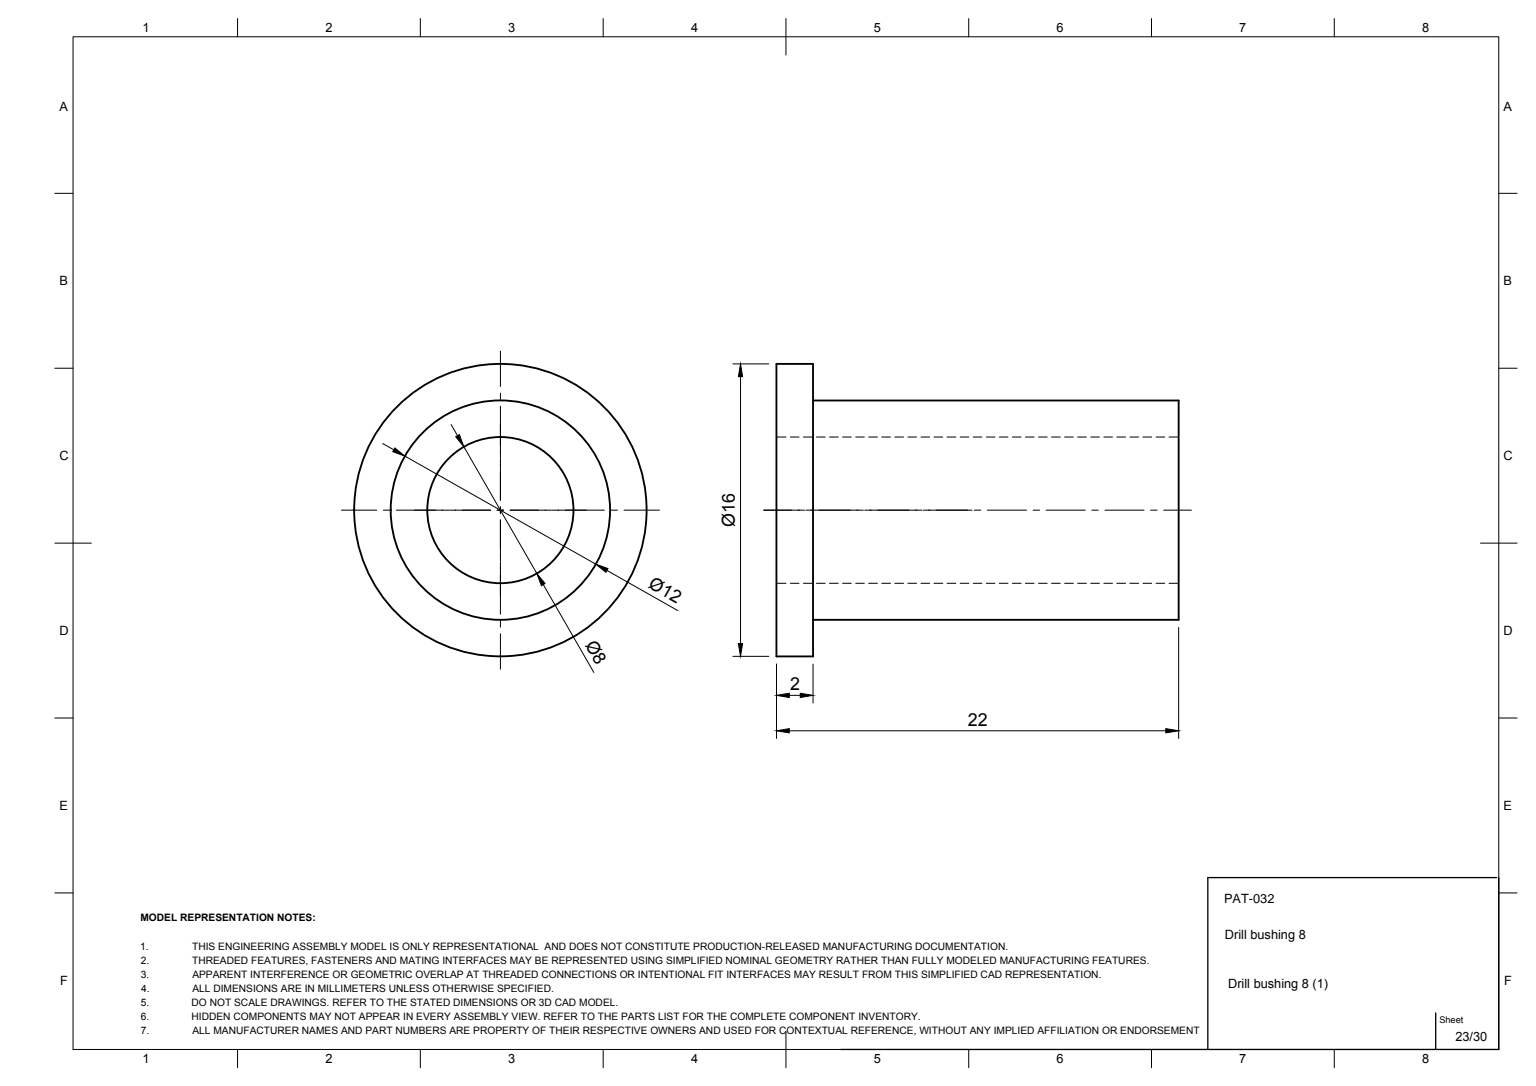
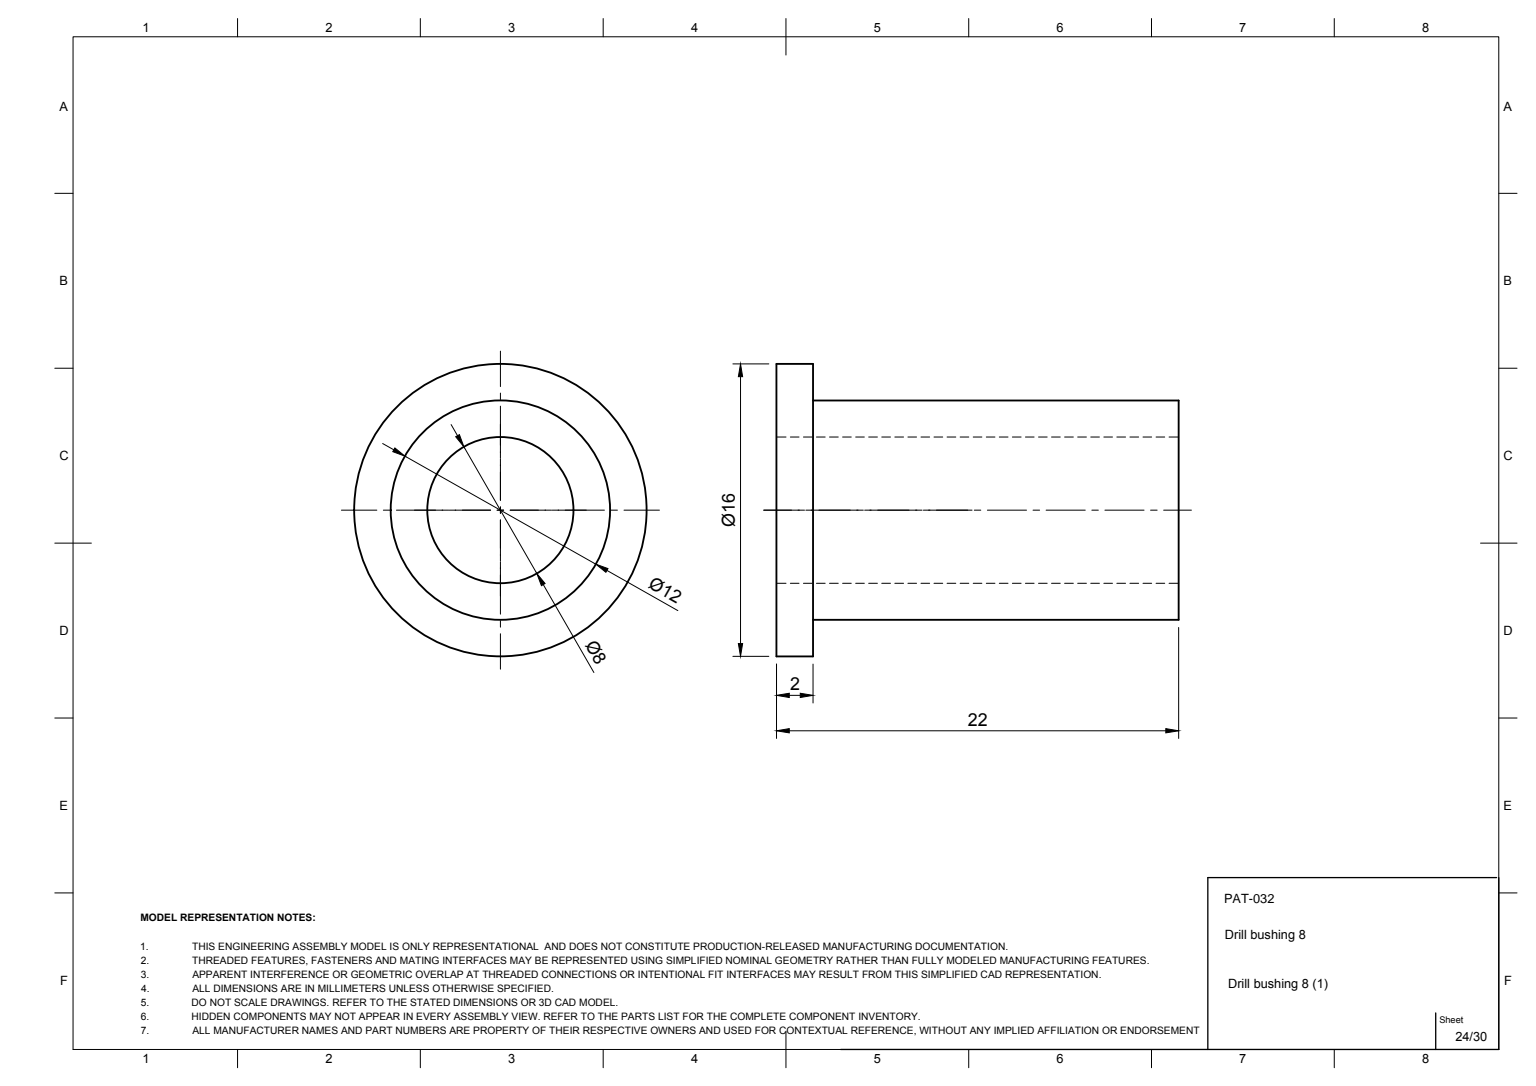
ISO-10303-21;
HEADER;
/* Generated by software containing ST-Developer
 * from STEP Tools, Inc. (www.steptools.com) 
 */

FILE_DESCRIPTION(
/* description */ ('Drill jig with bushing plate'),
/* implementation_level */ '2;1');

FILE_NAME(
/* name */ 'Drill bushing 8.step',
/* time_stamp */ '2026-10-27T10:51:08-07:00',
/* author */ (''),
/* organization */ (''),
/* preprocessor_version */ 'ST-DEVELOPER v20.2',
/* originating_system */ 'Autodesk Translation Framework v15.17.0.0',
/* authorisation */ '');

FILE_SCHEMA (('AUTOMOTIVE_DESIGN { 1 0 10303 214 3 1 1 }'));
ENDSEC;

DATA;
#10=MECHANICAL_DESIGN_GEOMETRIC_PRESENTATION_REPRESENTATION('',(#241),#6638);
#193=SHAPE_REPRESENTATION_RELATIONSHIP('SRR','None',#6758,#217);
#217=ADVANCED_BREP_SHAPE_REPRESENTATION('',(#263),#6631);
#241=STYLED_ITEM('',(#6957),#263);
#263=MANIFOLD_SOLID_BREP('Body1',#3610);
#355=FACE_BOUND('',#980,.T.);
#356=FACE_BOUND('',#983,.T.);
#357=FACE_BOUND('',#987,.T.);
#481=PLANE('',#4245);
#482=PLANE('',#4250);
#483=PLANE('',#4256);
#679=FACE_OUTER_BOUND('',#979,.T.);
#680=FACE_OUTER_BOUND('',#981,.T.);
#681=FACE_OUTER_BOUND('',#982,.T.);
#682=FACE_OUTER_BOUND('',#984,.T.);
#683=FACE_OUTER_BOUND('',#985,.T.);
#684=FACE_OUTER_BOUND('',#986,.T.);
#979=EDGE_LOOP('',(#3185));
#980=EDGE_LOOP('',(#3186));
#981=EDGE_LOOP('',(#3187,#3188,#3189,#3190));
#982=EDGE_LOOP('',(#3191));
#983=EDGE_LOOP('',(#3192));
#984=EDGE_LOOP('',(#3193,#3194,#3195,#3196));
#985=EDGE_LOOP('',(#3197,#3198,#3199,#3200));
#986=EDGE_LOOP('',(#3201));
#987=EDGE_LOOP('',(#3202));
#1266=LINE('',#6442,#1527);
#1267=LINE('',#6448,#1528);
#1268=LINE('',#6452,#1529);
#1527=VECTOR('',#5303,0.8);
#1528=VECTOR('',#5310,0.4);
#1529=VECTOR('',#5315,0.6);
#1688=CIRCLE('',#4246,0.8);
#1689=CIRCLE('',#4247,0.6);
#1690=CIRCLE('',#4249,0.8);
#1691=CIRCLE('',#4251,0.4);
#1692=CIRCLE('',#4253,0.4);
#1693=CIRCLE('',#4255,0.6);
#1968=VERTEX_POINT('',#6435);
#1969=VERTEX_POINT('',#6437);
#1970=VERTEX_POINT('',#6440);
#1971=VERTEX_POINT('',#6444);
#1972=VERTEX_POINT('',#6447);
#1973=VERTEX_POINT('',#6451);
#2380=EDGE_CURVE('',#1968,#1968,#1688,.T.);
#2381=EDGE_CURVE('',#1969,#1969,#1689,.T.);
#2382=EDGE_CURVE('',#1970,#1970,#1690,.T.);
#2383=EDGE_CURVE('',#1970,#1968,#1266,.T.);
#2384=EDGE_CURVE('',#1971,#1971,#1691,.T.);
#2385=EDGE_CURVE('',#1971,#1972,#1267,.T.);
#2386=EDGE_CURVE('',#1972,#1972,#1692,.T.);
#2387=EDGE_CURVE('',#1969,#1973,#1268,.T.);
#2388=EDGE_CURVE('',#1973,#1973,#1693,.T.);
#3185=ORIENTED_EDGE('',*,*,#2380,.F.);
#3186=ORIENTED_EDGE('',*,*,#2381,.T.);
#3187=ORIENTED_EDGE('',*,*,#2382,.F.);
#3188=ORIENTED_EDGE('',*,*,#2383,.T.);
#3189=ORIENTED_EDGE('',*,*,#2380,.T.);
#3190=ORIENTED_EDGE('',*,*,#2383,.F.);
#3191=ORIENTED_EDGE('',*,*,#2382,.T.);
#3192=ORIENTED_EDGE('',*,*,#2384,.T.);
#3193=ORIENTED_EDGE('',*,*,#2384,.F.);
#3194=ORIENTED_EDGE('',*,*,#2385,.T.);
#3195=ORIENTED_EDGE('',*,*,#2386,.T.);
#3196=ORIENTED_EDGE('',*,*,#2385,.F.);
#3197=ORIENTED_EDGE('',*,*,#2381,.F.);
#3198=ORIENTED_EDGE('',*,*,#2387,.T.);
#3199=ORIENTED_EDGE('',*,*,#2388,.T.);
#3200=ORIENTED_EDGE('',*,*,#2387,.F.);
#3201=ORIENTED_EDGE('',*,*,#2388,.F.);
#3202=ORIENTED_EDGE('',*,*,#2386,.F.);
#3360=CYLINDRICAL_SURFACE('',#4248,0.8);
#3361=CYLINDRICAL_SURFACE('',#4252,0.4);
#3362=CYLINDRICAL_SURFACE('',#4254,0.6);
#3554=ADVANCED_FACE('',(#679,#355),#481,.F.);
#3555=ADVANCED_FACE('',(#680),#3360,.T.);
#3556=ADVANCED_FACE('',(#681,#356),#482,.T.);
#3557=ADVANCED_FACE('',(#682),#3361,.F.);
#3558=ADVANCED_FACE('',(#683),#3362,.T.);
#3559=ADVANCED_FACE('',(#684,#357),#483,.F.);
#3610=CLOSED_SHELL('',(#3554,#3555,#3556,#3557,#3558,#3559));
#4244=AXIS2_PLACEMENT_3D('',#6433,#5291,#5292);
#4245=AXIS2_PLACEMENT_3D('',#6434,#5293,#5294);
#4246=AXIS2_PLACEMENT_3D('',#6436,#5295,#5296);
#4247=AXIS2_PLACEMENT_3D('',#6438,#5297,#5298);
#4248=AXIS2_PLACEMENT_3D('',#6439,#5299,#5300);
#4249=AXIS2_PLACEMENT_3D('',#6441,#5301,#5302);
#4250=AXIS2_PLACEMENT_3D('',#6443,#5304,#5305);
#4251=AXIS2_PLACEMENT_3D('',#6445,#5306,#5307);
#4252=AXIS2_PLACEMENT_3D('',#6446,#5308,#5309);
#4253=AXIS2_PLACEMENT_3D('',#6449,#5311,#5312);
#4254=AXIS2_PLACEMENT_3D('',#6450,#5313,#5314);
#4255=AXIS2_PLACEMENT_3D('',#6453,#5316,#5317);
#4256=AXIS2_PLACEMENT_3D('',#6454,#5318,#5319);
#5291=DIRECTION('axis',(0.,0.,1.));
#5292=DIRECTION('refdir',(1.,0.,0.));
#5293=DIRECTION('center_axis',(0.,0.,1.));
#5294=DIRECTION('ref_axis',(1.,0.,0.));
#5295=DIRECTION('center_axis',(0.,0.,1.));
#5296=DIRECTION('ref_axis',(1.,0.,0.));
#5297=DIRECTION('center_axis',(0.,0.,1.));
#5298=DIRECTION('ref_axis',(1.,0.,0.));
#5299=DIRECTION('center_axis',(0.,0.,1.));
#5300=DIRECTION('ref_axis',(1.,0.,0.));
#5301=DIRECTION('center_axis',(0.,0.,1.));
#5302=DIRECTION('ref_axis',(1.,0.,0.));
#5303=DIRECTION('',(0.,0.,-1.));
#5304=DIRECTION('center_axis',(0.,0.,1.));
#5305=DIRECTION('ref_axis',(1.,0.,0.));
#5306=DIRECTION('center_axis',(0.,0.,-1.));
#5307=DIRECTION('ref_axis',(1.,0.,0.));
#5308=DIRECTION('center_axis',(0.,0.,1.));
#5309=DIRECTION('ref_axis',(1.,0.,0.));
#5310=DIRECTION('',(0.,0.,-1.));
#5311=DIRECTION('center_axis',(0.,0.,-1.));
#5312=DIRECTION('ref_axis',(1.,0.,0.));
#5313=DIRECTION('center_axis',(0.,0.,1.));
#5314=DIRECTION('ref_axis',(1.,0.,0.));
#5315=DIRECTION('',(0.,0.,-1.));
#5316=DIRECTION('center_axis',(0.,0.,1.));
#5317=DIRECTION('ref_axis',(1.,0.,0.));
#5318=DIRECTION('center_axis',(0.,0.,1.));
#5319=DIRECTION('ref_axis',(1.,0.,0.));
#6433=CARTESIAN_POINT('',(0.,0.,0.));
#6434=CARTESIAN_POINT('Origin',(-2.,-1.,4.5));
#6435=CARTESIAN_POINT('',(-2.8,-1.,4.5));
#6436=CARTESIAN_POINT('Origin',(-2.,-1.,4.5));
#6437=CARTESIAN_POINT('',(-2.6,-1.,4.5));
#6438=CARTESIAN_POINT('Origin',(-2.,-1.,4.5));
#6439=CARTESIAN_POINT('Origin',(-2.,-1.,4.5));
#6440=CARTESIAN_POINT('',(-2.8,-1.,4.7));
#6441=CARTESIAN_POINT('Origin',(-2.,-1.,4.7));
#6442=CARTESIAN_POINT('',(-2.8,-1.,4.5));
#6443=CARTESIAN_POINT('Origin',(-2.,-1.,4.7));
#6444=CARTESIAN_POINT('',(-2.4,-1.,4.7));
#6445=CARTESIAN_POINT('Origin',(-2.,-1.,4.7));
#6446=CARTESIAN_POINT('Origin',(-2.,-1.,2.5));
#6447=CARTESIAN_POINT('',(-2.4,-1.,2.5));
#6448=CARTESIAN_POINT('',(-2.4,-1.,2.5));
#6449=CARTESIAN_POINT('Origin',(-2.,-1.,2.5));
#6450=CARTESIAN_POINT('Origin',(-2.,-1.,2.5));
#6451=CARTESIAN_POINT('',(-2.6,-1.,2.5));
#6452=CARTESIAN_POINT('',(-2.6,-1.,2.5));
#6453=CARTESIAN_POINT('Origin',(-2.,-1.,2.5));
#6454=CARTESIAN_POINT('Origin',(-2.,-1.,2.5));
#6602=UNCERTAINTY_MEASURE_WITH_UNIT(LENGTH_MEASURE(0.001),#6639,
'DISTANCE_ACCURACY_VALUE',
'Maximum model space distance between geometric entities at asserted c
onnectivities');
#6609=UNCERTAINTY_MEASURE_WITH_UNIT(LENGTH_MEASURE(0.001),#6639,
'DISTANCE_ACCURACY_VALUE',
'Maximum model space distance between geometric entities at asserted c
onnectivities');
#6631=(
GEOMETRIC_REPRESENTATION_CONTEXT(3)
GLOBAL_UNCERTAINTY_ASSIGNED_CONTEXT((#6602))
GLOBAL_UNIT_ASSIGNED_CONTEXT((#6639,#6641,#6642))
REPRESENTATION_CONTEXT('','3D')
);
#6638=(
GEOMETRIC_REPRESENTATION_CONTEXT(3)
GLOBAL_UNCERTAINTY_ASSIGNED_CONTEXT((#6609))
GLOBAL_UNIT_ASSIGNED_CONTEXT((#6639,#6641,#6642))
REPRESENTATION_CONTEXT('','3D')
);
#6639=(
LENGTH_UNIT()
NAMED_UNIT(*)
SI_UNIT(.CENTI.,.METRE.)
);
#6641=(
NAMED_UNIT(*)
PLANE_ANGLE_UNIT()
SI_UNIT($,.RADIAN.)
);
#6642=(
NAMED_UNIT(*)
SI_UNIT($,.STERADIAN.)
SOLID_ANGLE_UNIT()
);
#6664=SHAPE_DEFINITION_REPRESENTATION(#6720,#6758);
#6720=PRODUCT_DEFINITION_SHAPE('',$,#6787);
#6758=SHAPE_REPRESENTATION('',(#4244),#6631);
#6765=PRODUCT_DEFINITION_CONTEXT('part definition',#6851,'design');
#6787=PRODUCT_DEFINITION('Drill bushing 8','Drill bushing 8',#6815,#6765);
#6815=PRODUCT_DEFINITION_FORMATION('',$,#6874);
#6851=APPLICATION_CONTEXT(
'Core Data for Automotive Mechanical Design Process');
#6852=PRODUCT_CONTEXT('part definition',#6851,'mechanical');
#6874=PRODUCT('Drill bushing 8','Drill bushing 8','Drill bushing 8',(#6852));
#6951=COLOUR_RGB('Off White',0.89,0.88,0.83);
#6952=FILL_AREA_STYLE_COLOUR('',#6951);
#6953=FILL_AREA_STYLE('',(#6952));
#6954=SURFACE_STYLE_FILL_AREA(#6953);
#6955=SURFACE_SIDE_STYLE('',(#6954));
#6956=SURFACE_STYLE_USAGE(.BOTH.,#6955);
#6957=PRESENTATION_STYLE_ASSIGNMENT((#6956));
ENDSEC;
END-ISO-10303-21;
